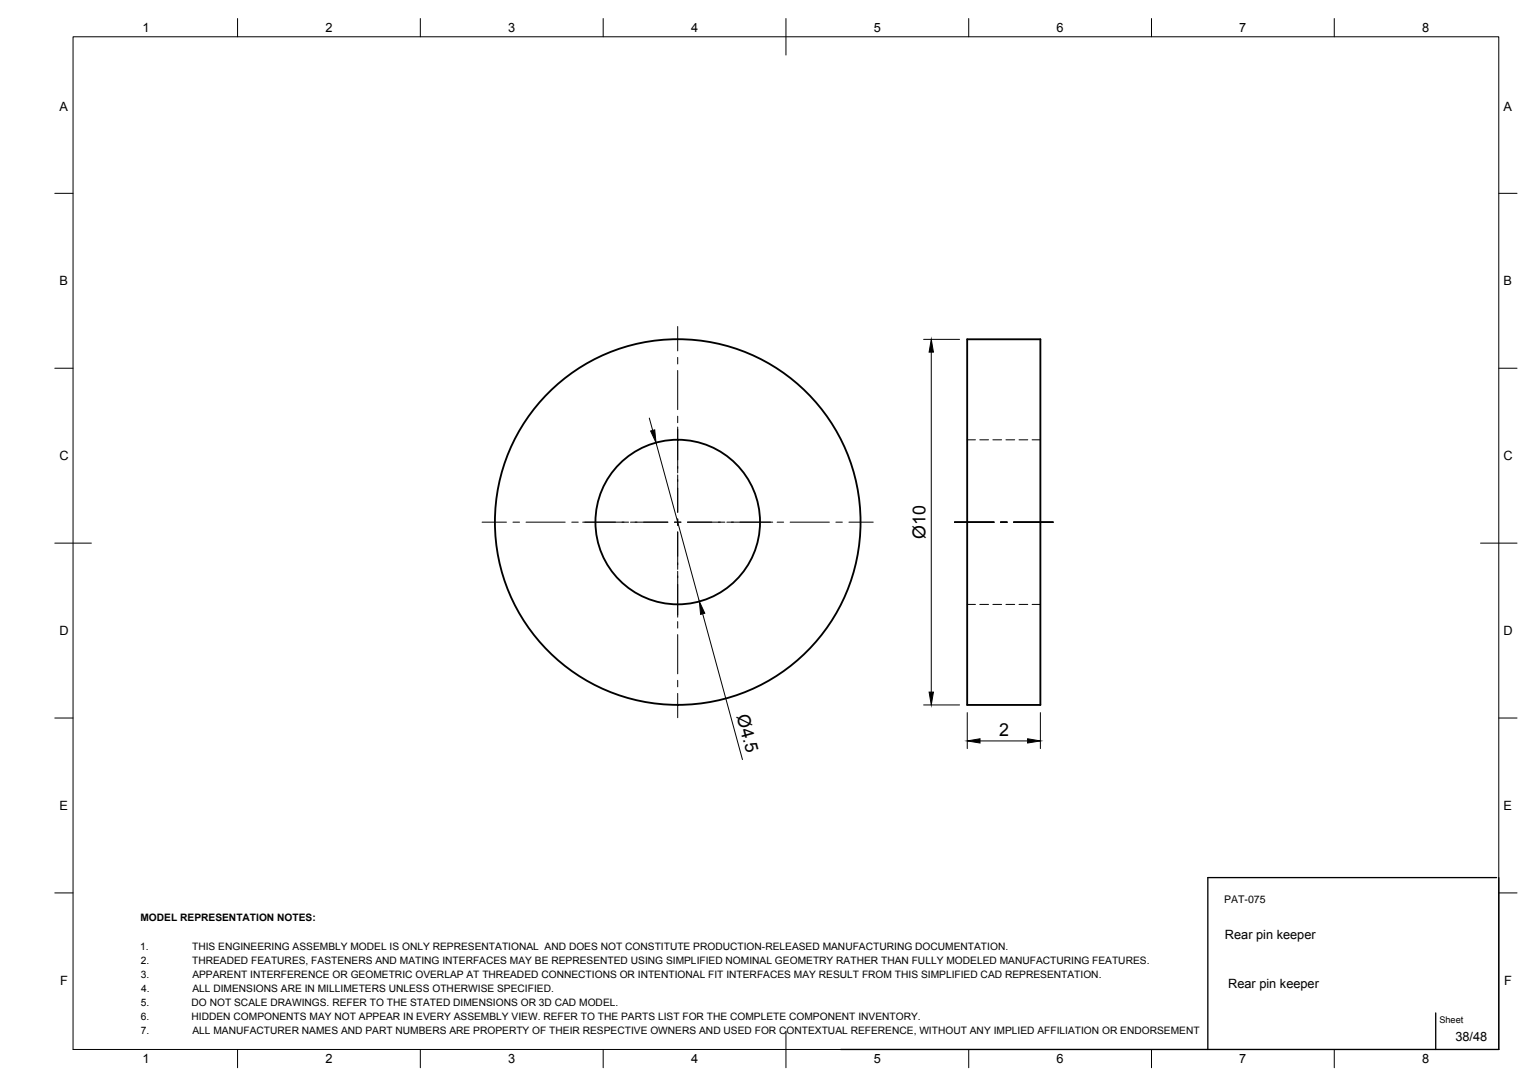
ISO-10303-21;
HEADER;
/* Generated by software containing ST-Developer
 * from STEP Tools, Inc. (www.steptools.com) 
 */

FILE_DESCRIPTION(
/* description */ ('Over-Centre Plunger Toggle Clamp on Slotted Fixture Frame'),
/* implementation_level */ '2;1');

FILE_NAME(
/* name */ 
'Rear pin keeper.step',
/* time_stamp */ '2026-10-28T03:23:24-07:00',
/* author */ (''),
/* organization */ (''),
/* preprocessor_version */ 'ST-DEVELOPER v20.2',
/* originating_system */ 'Autodesk Translation Framework v15.17.0.0',
/* authorisation */ '');

FILE_SCHEMA (('AUTOMOTIVE_DESIGN { 1 0 10303 214 3 1 1 }'));
ENDSEC;

DATA;
#10=MECHANICAL_DESIGN_GEOMETRIC_PRESENTATION_REPRESENTATION('',(#552),#15212);
#460=SHAPE_REPRESENTATION_RELATIONSHIP('SRR','None',#15437,#502);
#502=ADVANCED_BREP_SHAPE_REPRESENTATION('',(#601),#15199);
#552=STYLED_ITEM('',(#15719),#601);
#601=MANIFOLD_SOLID_BREP('Body1',#8286);
#763=FACE_BOUND('',#2106,.T.);
#764=FACE_BOUND('',#2108,.T.);
#1013=PLANE('',#9498);
#1014=PLANE('',#9499);
#1465=FACE_OUTER_BOUND('',#2103,.T.);
#1466=FACE_OUTER_BOUND('',#2104,.T.);
#1467=FACE_OUTER_BOUND('',#2105,.T.);
#1468=FACE_OUTER_BOUND('',#2107,.T.);
#2103=EDGE_LOOP('',(#7195,#7196,#7197,#7198));
#2104=EDGE_LOOP('',(#7199,#7200,#7201,#7202));
#2105=EDGE_LOOP('',(#7203));
#2106=EDGE_LOOP('',(#7204));
#2107=EDGE_LOOP('',(#7205));
#2108=EDGE_LOOP('',(#7206));
#2715=LINE('',#14552,#3345);
#2716=LINE('',#14558,#3346);
#3345=VECTOR('',#11700,0.225);
#3346=VECTOR('',#11707,0.5);
#3796=CIRCLE('',#9493,0.225);
#3797=CIRCLE('',#9494,0.225);
#3798=CIRCLE('',#9496,0.5);
#3799=CIRCLE('',#9497,0.5);
#4408=VERTEX_POINT('',#14549);
#4409=VERTEX_POINT('',#14551);
#4410=VERTEX_POINT('',#14555);
#4411=VERTEX_POINT('',#14557);
#5358=EDGE_CURVE('',#4408,#4408,#3796,.T.);
#5359=EDGE_CURVE('',#4408,#4409,#2715,.T.);
#5360=EDGE_CURVE('',#4409,#4409,#3797,.T.);
#5361=EDGE_CURVE('',#4410,#4410,#3798,.T.);
#5362=EDGE_CURVE('',#4410,#4411,#2716,.T.);
#5363=EDGE_CURVE('',#4411,#4411,#3799,.T.);
#7195=ORIENTED_EDGE('',*,*,#5358,.F.);
#7196=ORIENTED_EDGE('',*,*,#5359,.T.);
#7197=ORIENTED_EDGE('',*,*,#5360,.T.);
#7198=ORIENTED_EDGE('',*,*,#5359,.F.);
#7199=ORIENTED_EDGE('',*,*,#5361,.F.);
#7200=ORIENTED_EDGE('',*,*,#5362,.T.);
#7201=ORIENTED_EDGE('',*,*,#5363,.T.);
#7202=ORIENTED_EDGE('',*,*,#5362,.F.);
#7203=ORIENTED_EDGE('',*,*,#5361,.T.);
#7204=ORIENTED_EDGE('',*,*,#5358,.T.);
#7205=ORIENTED_EDGE('',*,*,#5363,.F.);
#7206=ORIENTED_EDGE('',*,*,#5360,.F.);
#7735=CYLINDRICAL_SURFACE('',#9492,0.225);
#7736=CYLINDRICAL_SURFACE('',#9495,0.5);
#8137=ADVANCED_FACE('',(#1465),#7735,.F.);
#8138=ADVANCED_FACE('',(#1466),#7736,.T.);
#8139=ADVANCED_FACE('',(#1467,#763),#1013,.T.);
#8140=ADVANCED_FACE('',(#1468,#764),#1014,.F.);
#8286=CLOSED_SHELL('',(#8137,#8138,#8139,#8140));
#9491=AXIS2_PLACEMENT_3D('',#14547,#11694,#11695);
#9492=AXIS2_PLACEMENT_3D('',#14548,#11696,#11697);
#9493=AXIS2_PLACEMENT_3D('',#14550,#11698,#11699);
#9494=AXIS2_PLACEMENT_3D('',#14553,#11701,#11702);
#9495=AXIS2_PLACEMENT_3D('',#14554,#11703,#11704);
#9496=AXIS2_PLACEMENT_3D('',#14556,#11705,#11706);
#9497=AXIS2_PLACEMENT_3D('',#14559,#11708,#11709);
#9498=AXIS2_PLACEMENT_3D('',#14560,#11710,#11711);
#9499=AXIS2_PLACEMENT_3D('',#14561,#11712,#11713);
#11694=DIRECTION('axis',(0.,0.,1.));
#11695=DIRECTION('refdir',(1.,0.,0.));
#11696=DIRECTION('center_axis',(0.,1.,0.));
#11697=DIRECTION('ref_axis',(1.,0.,0.));
#11698=DIRECTION('center_axis',(0.,-1.,0.));
#11699=DIRECTION('ref_axis',(1.,0.,0.));
#11700=DIRECTION('',(0.,-1.,0.));
#11701=DIRECTION('center_axis',(0.,-1.,0.));
#11702=DIRECTION('ref_axis',(1.,0.,0.));
#11703=DIRECTION('center_axis',(0.,1.,0.));
#11704=DIRECTION('ref_axis',(1.,0.,0.));
#11705=DIRECTION('center_axis',(0.,1.,0.));
#11706=DIRECTION('ref_axis',(1.,0.,0.));
#11707=DIRECTION('',(0.,-1.,0.));
#11708=DIRECTION('center_axis',(0.,1.,0.));
#11709=DIRECTION('ref_axis',(1.,0.,0.));
#11710=DIRECTION('center_axis',(0.,1.,0.));
#11711=DIRECTION('ref_axis',(1.,0.,0.));
#11712=DIRECTION('center_axis',(0.,1.,0.));
#11713=DIRECTION('ref_axis',(1.,0.,0.));
#14547=CARTESIAN_POINT('',(0.,0.,0.));
#14548=CARTESIAN_POINT('Origin',(-2.82632109303527,-2.7,8.79263101785268));
#14549=CARTESIAN_POINT('',(-3.05132109303527,-2.5,8.79263101785268));
#14550=CARTESIAN_POINT('Origin',(-2.82632109303527,-2.5,8.79263101785268));
#14551=CARTESIAN_POINT('',(-3.05132109303527,-2.7,8.79263101785268));
#14552=CARTESIAN_POINT('',(-3.05132109303527,-2.7,8.79263101785268));
#14553=CARTESIAN_POINT('Origin',(-2.82632109303527,-2.7,8.79263101785268));
#14554=CARTESIAN_POINT('Origin',(-2.82632109303527,-2.7,8.79263101785268));
#14555=CARTESIAN_POINT('',(-3.32632109303527,-2.5,8.79263101785268));
#14556=CARTESIAN_POINT('Origin',(-2.82632109303527,-2.5,8.79263101785268));
#14557=CARTESIAN_POINT('',(-3.32632109303527,-2.7,8.79263101785268));
#14558=CARTESIAN_POINT('',(-3.32632109303527,-2.7,8.79263101785268));
#14559=CARTESIAN_POINT('Origin',(-2.82632109303527,-2.7,8.79263101785268));
#14560=CARTESIAN_POINT('Origin',(-2.82632109303527,-2.5,8.79263101785268));
#14561=CARTESIAN_POINT('Origin',(-2.82632109303527,-2.7,8.79263101785268));
#15149=UNCERTAINTY_MEASURE_WITH_UNIT(LENGTH_MEASURE(0.001),#15213,
'DISTANCE_ACCURACY_VALUE',
'Maximum model space distance between geometric entities at asserted c
onnectivities');
#15162=UNCERTAINTY_MEASURE_WITH_UNIT(LENGTH_MEASURE(0.001),#15213,
'DISTANCE_ACCURACY_VALUE',
'Maximum model space distance between geometric entities at asserted c
onnectivities');
#15199=(
GEOMETRIC_REPRESENTATION_CONTEXT(3)
GLOBAL_UNCERTAINTY_ASSIGNED_CONTEXT((#15149))
GLOBAL_UNIT_ASSIGNED_CONTEXT((#15213,#15215,#15216))
REPRESENTATION_CONTEXT('','3D')
);
#15212=(
GEOMETRIC_REPRESENTATION_CONTEXT(3)
GLOBAL_UNCERTAINTY_ASSIGNED_CONTEXT((#15162))
GLOBAL_UNIT_ASSIGNED_CONTEXT((#15213,#15215,#15216))
REPRESENTATION_CONTEXT('','3D')
);
#15213=(
LENGTH_UNIT()
NAMED_UNIT(*)
SI_UNIT(.CENTI.,.METRE.)
);
#15215=(
NAMED_UNIT(*)
PLANE_ANGLE_UNIT()
SI_UNIT($,.RADIAN.)
);
#15216=(
NAMED_UNIT(*)
SI_UNIT($,.STERADIAN.)
SOLID_ANGLE_UNIT()
);
#15253=SHAPE_DEFINITION_REPRESENTATION(#15309,#15437);
#15309=PRODUCT_DEFINITION_SHAPE('',$,#15487);
#15437=SHAPE_REPRESENTATION('',(#9491),#15199);
#15450=PRODUCT_DEFINITION_CONTEXT('part definition',#15599,'design');
#15487=PRODUCT_DEFINITION('Rear pin keeper','Rear pin keeper',#15536,#15450);
#15536=PRODUCT_DEFINITION_FORMATION('',$,#15637);
#15599=APPLICATION_CONTEXT(
'Core Data for Automotive Mechanical Design Process');
#15600=PRODUCT_CONTEXT('part definition',#15599,'mechanical');
#15637=PRODUCT('Rear pin keeper','Rear pin keeper','Rear pin keeper',(#15600));
#15713=COLOUR_RGB('Grey',0.48,0.52,0.57);
#15714=FILL_AREA_STYLE_COLOUR('',#15713);
#15715=FILL_AREA_STYLE('',(#15714));
#15716=SURFACE_STYLE_FILL_AREA(#15715);
#15717=SURFACE_SIDE_STYLE('',(#15716));
#15718=SURFACE_STYLE_USAGE(.BOTH.,#15717);
#15719=PRESENTATION_STYLE_ASSIGNMENT((#15718));
ENDSEC;
END-ISO-10303-21;
